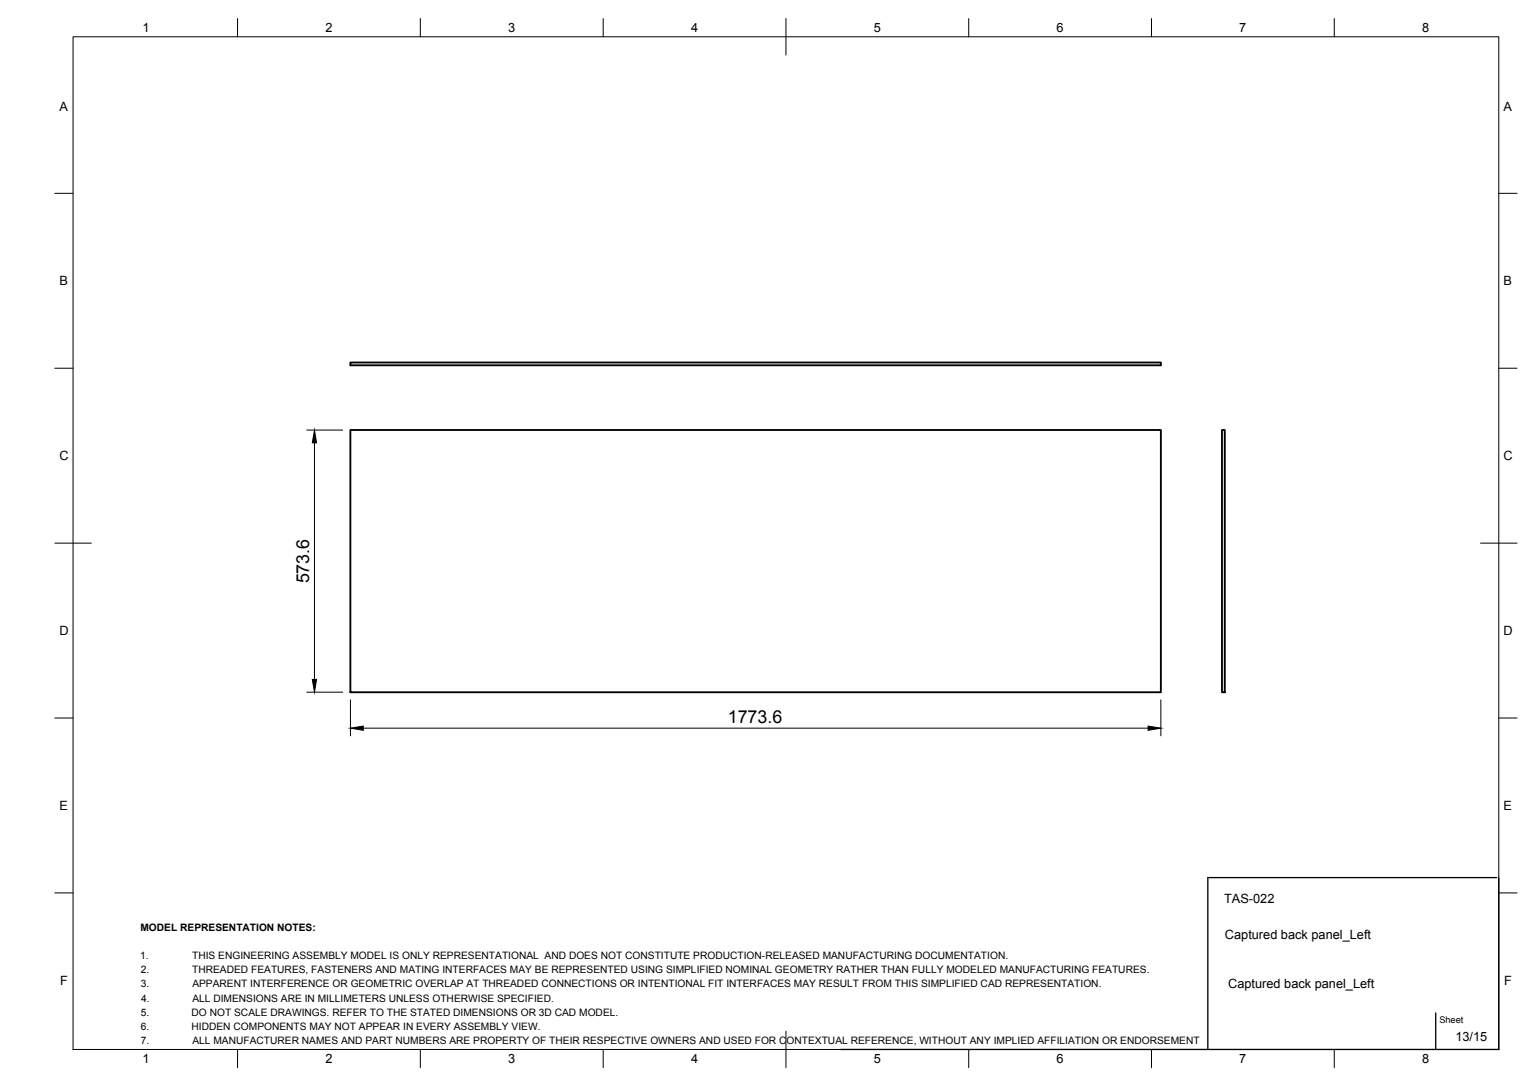
ISO-10303-21;
HEADER;
/* Generated by software containing ST-Developer
 * from STEP Tools, Inc. (www.steptools.com) 
 */

FILE_DESCRIPTION(
/* description */ (''),
/* implementation_level */ '2;1');

FILE_NAME(
/* name */ 'Captured back panel_Left.step',
/* time_stamp */ '2026-11-15T21:02:08-08:00',
/* author */ (''),
/* organization */ (''),
/* preprocessor_version */ 'ST-DEVELOPER v20.2',
/* originating_system */ 'Autodesk Translation Framework v15.17.0.0',
/* authorisation */ '');

FILE_SCHEMA (('AUTOMOTIVE_DESIGN { 1 0 10303 214 3 1 1 }'));
ENDSEC;

DATA;
#10=MECHANICAL_DESIGN_GEOMETRIC_PRESENTATION_REPRESENTATION('',(#607),#31566);
#577=SHAPE_REPRESENTATION_RELATIONSHIP('SRR','None',#31641,#592);
#592=ADVANCED_BREP_SHAPE_REPRESENTATION('',(#622),#31556);
#607=STYLED_ITEM('',(#31720),#622);
#622=MANIFOLD_SOLID_BREP('Body1',#5720);
#691=FACE_OUTER_BOUND('',#980,.T.);
#692=FACE_OUTER_BOUND('',#981,.T.);
#693=FACE_OUTER_BOUND('',#982,.T.);
#694=FACE_OUTER_BOUND('',#983,.T.);
#695=FACE_OUTER_BOUND('',#984,.T.);
#696=FACE_OUTER_BOUND('',#985,.T.);
#980=EDGE_LOOP('',(#3921,#3922,#3923,#3924));
#981=EDGE_LOOP('',(#3925,#3926,#3927,#3928));
#982=EDGE_LOOP('',(#3929,#3930,#3931,#3932));
#983=EDGE_LOOP('',(#3933,#3934,#3935,#3936));
#984=EDGE_LOOP('',(#3937,#3938,#3939,#3940));
#985=EDGE_LOOP('',(#3941,#3942,#3943,#3944));
#1313=LINE('',#7875,#1820);
#1314=LINE('',#7877,#1821);
#1315=LINE('',#7879,#1822);
#1316=LINE('',#7880,#1823);
#1317=LINE('',#7883,#1824);
#1318=LINE('',#7885,#1825);
#1319=LINE('',#7886,#1826);
#1320=LINE('',#7889,#1827);
#1321=LINE('',#7891,#1828);
#1322=LINE('',#7892,#1829);
#1323=LINE('',#7894,#1830);
#1324=LINE('',#7895,#1831);
#1820=VECTOR('',#6603,1.);
#1821=VECTOR('',#6604,1.);
#1822=VECTOR('',#6605,1.);
#1823=VECTOR('',#6606,1.);
#1824=VECTOR('',#6609,1.);
#1825=VECTOR('',#6610,1.);
#1826=VECTOR('',#6611,1.);
#1827=VECTOR('',#6614,1.);
#1828=VECTOR('',#6615,1.);
#1829=VECTOR('',#6616,1.);
#1830=VECTOR('',#6619,1.);
#1831=VECTOR('',#6620,1.);
#2318=VERTEX_POINT('',#7873);
#2319=VERTEX_POINT('',#7874);
#2320=VERTEX_POINT('',#7876);
#2321=VERTEX_POINT('',#7878);
#2322=VERTEX_POINT('',#7882);
#2323=VERTEX_POINT('',#7884);
#2324=VERTEX_POINT('',#7888);
#2325=VERTEX_POINT('',#7890);
#2956=EDGE_CURVE('',#2318,#2319,#1313,.T.);
#2957=EDGE_CURVE('',#2319,#2320,#1314,.T.);
#2958=EDGE_CURVE('',#2321,#2320,#1315,.T.);
#2959=EDGE_CURVE('',#2318,#2321,#1316,.T.);
#2960=EDGE_CURVE('',#2322,#2318,#1317,.T.);
#2961=EDGE_CURVE('',#2323,#2321,#1318,.T.);
#2962=EDGE_CURVE('',#2322,#2323,#1319,.T.);
#2963=EDGE_CURVE('',#2324,#2322,#1320,.T.);
#2964=EDGE_CURVE('',#2325,#2323,#1321,.T.);
#2965=EDGE_CURVE('',#2324,#2325,#1322,.T.);
#2966=EDGE_CURVE('',#2319,#2324,#1323,.T.);
#2967=EDGE_CURVE('',#2320,#2325,#1324,.T.);
#3921=ORIENTED_EDGE('',*,*,#2956,.T.);
#3922=ORIENTED_EDGE('',*,*,#2957,.T.);
#3923=ORIENTED_EDGE('',*,*,#2958,.F.);
#3924=ORIENTED_EDGE('',*,*,#2959,.F.);
#3925=ORIENTED_EDGE('',*,*,#2960,.T.);
#3926=ORIENTED_EDGE('',*,*,#2959,.T.);
#3927=ORIENTED_EDGE('',*,*,#2961,.F.);
#3928=ORIENTED_EDGE('',*,*,#2962,.F.);
#3929=ORIENTED_EDGE('',*,*,#2963,.T.);
#3930=ORIENTED_EDGE('',*,*,#2962,.T.);
#3931=ORIENTED_EDGE('',*,*,#2964,.F.);
#3932=ORIENTED_EDGE('',*,*,#2965,.F.);
#3933=ORIENTED_EDGE('',*,*,#2966,.T.);
#3934=ORIENTED_EDGE('',*,*,#2965,.T.);
#3935=ORIENTED_EDGE('',*,*,#2967,.F.);
#3936=ORIENTED_EDGE('',*,*,#2957,.F.);
#3937=ORIENTED_EDGE('',*,*,#2967,.T.);
#3938=ORIENTED_EDGE('',*,*,#2964,.T.);
#3939=ORIENTED_EDGE('',*,*,#2961,.T.);
#3940=ORIENTED_EDGE('',*,*,#2958,.T.);
#3941=ORIENTED_EDGE('',*,*,#2966,.F.);
#3942=ORIENTED_EDGE('',*,*,#2956,.F.);
#3943=ORIENTED_EDGE('',*,*,#2960,.F.);
#3944=ORIENTED_EDGE('',*,*,#2963,.F.);
#5302=PLANE('',#6002);
#5303=PLANE('',#6003);
#5304=PLANE('',#6004);
#5305=PLANE('',#6005);
#5306=PLANE('',#6006);
#5307=PLANE('',#6007);
#5505=ADVANCED_FACE('',(#691),#5302,.T.);
#5506=ADVANCED_FACE('',(#692),#5303,.T.);
#5507=ADVANCED_FACE('',(#693),#5304,.T.);
#5508=ADVANCED_FACE('',(#694),#5305,.T.);
#5509=ADVANCED_FACE('',(#695),#5306,.T.);
#5510=ADVANCED_FACE('',(#696),#5307,.F.);
#5720=CLOSED_SHELL('',(#5505,#5506,#5507,#5508,#5509,#5510));
#6001=AXIS2_PLACEMENT_3D('',#7871,#6599,#6600);
#6002=AXIS2_PLACEMENT_3D('',#7872,#6601,#6602);
#6003=AXIS2_PLACEMENT_3D('',#7881,#6607,#6608);
#6004=AXIS2_PLACEMENT_3D('',#7887,#6612,#6613);
#6005=AXIS2_PLACEMENT_3D('',#7893,#6617,#6618);
#6006=AXIS2_PLACEMENT_3D('',#7896,#6621,#6622);
#6007=AXIS2_PLACEMENT_3D('',#7897,#6623,#6624);
#6599=DIRECTION('axis',(0.,0.,1.));
#6600=DIRECTION('refdir',(1.,0.,0.));
#6601=DIRECTION('center_axis',(0.,1.,0.));
#6602=DIRECTION('ref_axis',(-1.,0.,0.));
#6603=DIRECTION('',(-1.,0.,0.));
#6604=DIRECTION('',(0.,0.,1.));
#6605=DIRECTION('',(-1.,0.,0.));
#6606=DIRECTION('',(0.,0.,1.));
#6607=DIRECTION('center_axis',(1.,0.,0.));
#6608=DIRECTION('ref_axis',(0.,1.,0.));
#6609=DIRECTION('',(0.,1.,0.));
#6610=DIRECTION('',(0.,1.,0.));
#6611=DIRECTION('',(0.,0.,1.));
#6612=DIRECTION('center_axis',(0.,-1.,0.));
#6613=DIRECTION('ref_axis',(1.,0.,0.));
#6614=DIRECTION('',(1.,0.,0.));
#6615=DIRECTION('',(1.,0.,0.));
#6616=DIRECTION('',(0.,0.,1.));
#6617=DIRECTION('center_axis',(-1.,0.,0.));
#6618=DIRECTION('ref_axis',(0.,-1.,0.));
#6619=DIRECTION('',(0.,-1.,0.));
#6620=DIRECTION('',(0.,-1.,0.));
#6621=DIRECTION('center_axis',(0.,0.,1.));
#6622=DIRECTION('ref_axis',(1.,0.,0.));
#6623=DIRECTION('center_axis',(0.,0.,1.));
#6624=DIRECTION('ref_axis',(1.,0.,0.));
#7871=CARTESIAN_POINT('',(0.,0.,0.));
#7872=CARTESIAN_POINT('Origin',(57.36,0.6,0.));
#7873=CARTESIAN_POINT('',(57.36,0.6,0.));
#7874=CARTESIAN_POINT('',(0.,0.6,0.));
#7875=CARTESIAN_POINT('',(57.36,0.6,0.));
#7876=CARTESIAN_POINT('',(0.,0.6,177.36));
#7877=CARTESIAN_POINT('',(0.,0.6,0.));
#7878=CARTESIAN_POINT('',(57.36,0.6,177.36));
#7879=CARTESIAN_POINT('',(57.36,0.6,177.36));
#7880=CARTESIAN_POINT('',(57.36,0.6,0.));
#7881=CARTESIAN_POINT('Origin',(57.36,0.,0.));
#7882=CARTESIAN_POINT('',(57.36,0.,0.));
#7883=CARTESIAN_POINT('',(57.36,0.,0.));
#7884=CARTESIAN_POINT('',(57.36,0.,177.36));
#7885=CARTESIAN_POINT('',(57.36,0.,177.36));
#7886=CARTESIAN_POINT('',(57.36,0.,0.));
#7887=CARTESIAN_POINT('Origin',(0.,0.,0.));
#7888=CARTESIAN_POINT('',(0.,0.,0.));
#7889=CARTESIAN_POINT('',(0.,0.,0.));
#7890=CARTESIAN_POINT('',(0.,0.,177.36));
#7891=CARTESIAN_POINT('',(0.,0.,177.36));
#7892=CARTESIAN_POINT('',(0.,0.,0.));
#7893=CARTESIAN_POINT('Origin',(0.,0.6,0.));
#7894=CARTESIAN_POINT('',(0.,0.6,0.));
#7895=CARTESIAN_POINT('',(0.,0.6,177.36));
#7896=CARTESIAN_POINT('Origin',(28.68,0.3,177.36));
#7897=CARTESIAN_POINT('Origin',(28.68,0.3,0.));
#31539=UNCERTAINTY_MEASURE_WITH_UNIT(LENGTH_MEASURE(0.001),#31567,
'DISTANCE_ACCURACY_VALUE',
'Maximum model space distance between geometric entities at asserted c
onnectivities');
#31549=UNCERTAINTY_MEASURE_WITH_UNIT(LENGTH_MEASURE(0.001),#31567,
'DISTANCE_ACCURACY_VALUE',
'Maximum model space distance between geometric entities at asserted c
onnectivities');
#31556=(
GEOMETRIC_REPRESENTATION_CONTEXT(3)
GLOBAL_UNCERTAINTY_ASSIGNED_CONTEXT((#31539))
GLOBAL_UNIT_ASSIGNED_CONTEXT((#31567,#31569,#31570))
REPRESENTATION_CONTEXT('','3D')
);
#31566=(
GEOMETRIC_REPRESENTATION_CONTEXT(3)
GLOBAL_UNCERTAINTY_ASSIGNED_CONTEXT((#31549))
GLOBAL_UNIT_ASSIGNED_CONTEXT((#31567,#31569,#31570))
REPRESENTATION_CONTEXT('','3D')
);
#31567=(
LENGTH_UNIT()
NAMED_UNIT(*)
SI_UNIT(.CENTI.,.METRE.)
);
#31569=(
NAMED_UNIT(*)
PLANE_ANGLE_UNIT()
SI_UNIT($,.RADIAN.)
);
#31570=(
NAMED_UNIT(*)
SI_UNIT($,.STERADIAN.)
SOLID_ANGLE_UNIT()
);
#31577=SHAPE_DEFINITION_REPRESENTATION(#31593,#31641);
#31593=PRODUCT_DEFINITION_SHAPE('',$,#31658);
#31641=SHAPE_REPRESENTATION('',(#6001),#31556);
#31651=PRODUCT_DEFINITION_CONTEXT('part definition',#31701,'design');
#31658=PRODUCT_DEFINITION('Captured back panel_Left',
'Captured back panel_Left',#31674,#31651);
#31674=PRODUCT_DEFINITION_FORMATION('',$,#31709);
#31701=APPLICATION_CONTEXT(
'Core Data for Automotive Mechanical Design Process');
#31702=PRODUCT_CONTEXT('part definition',#31701,'mechanical');
#31709=PRODUCT('Captured back panel_Left','Captured back panel_Left',$,
(#31702));
#31720=PRESENTATION_STYLE_ASSIGNMENT((#31727));
#31727=SURFACE_STYLE_USAGE(.BOTH.,#31734);
#31734=SURFACE_SIDE_STYLE('',(#31741));
#31741=SURFACE_STYLE_FILL_AREA(#31748);
#31748=FILL_AREA_STYLE('Opaque(155,165,179)',(#31755));
#31755=FILL_AREA_STYLE_COLOUR('Opaque(155,165,179)',#31762);
#31762=COLOUR_RGB('Opaque(155,165,179)',0.607843137254902,0.647058823529412,
0.701960784313725);
ENDSEC;
END-ISO-10303-21;
